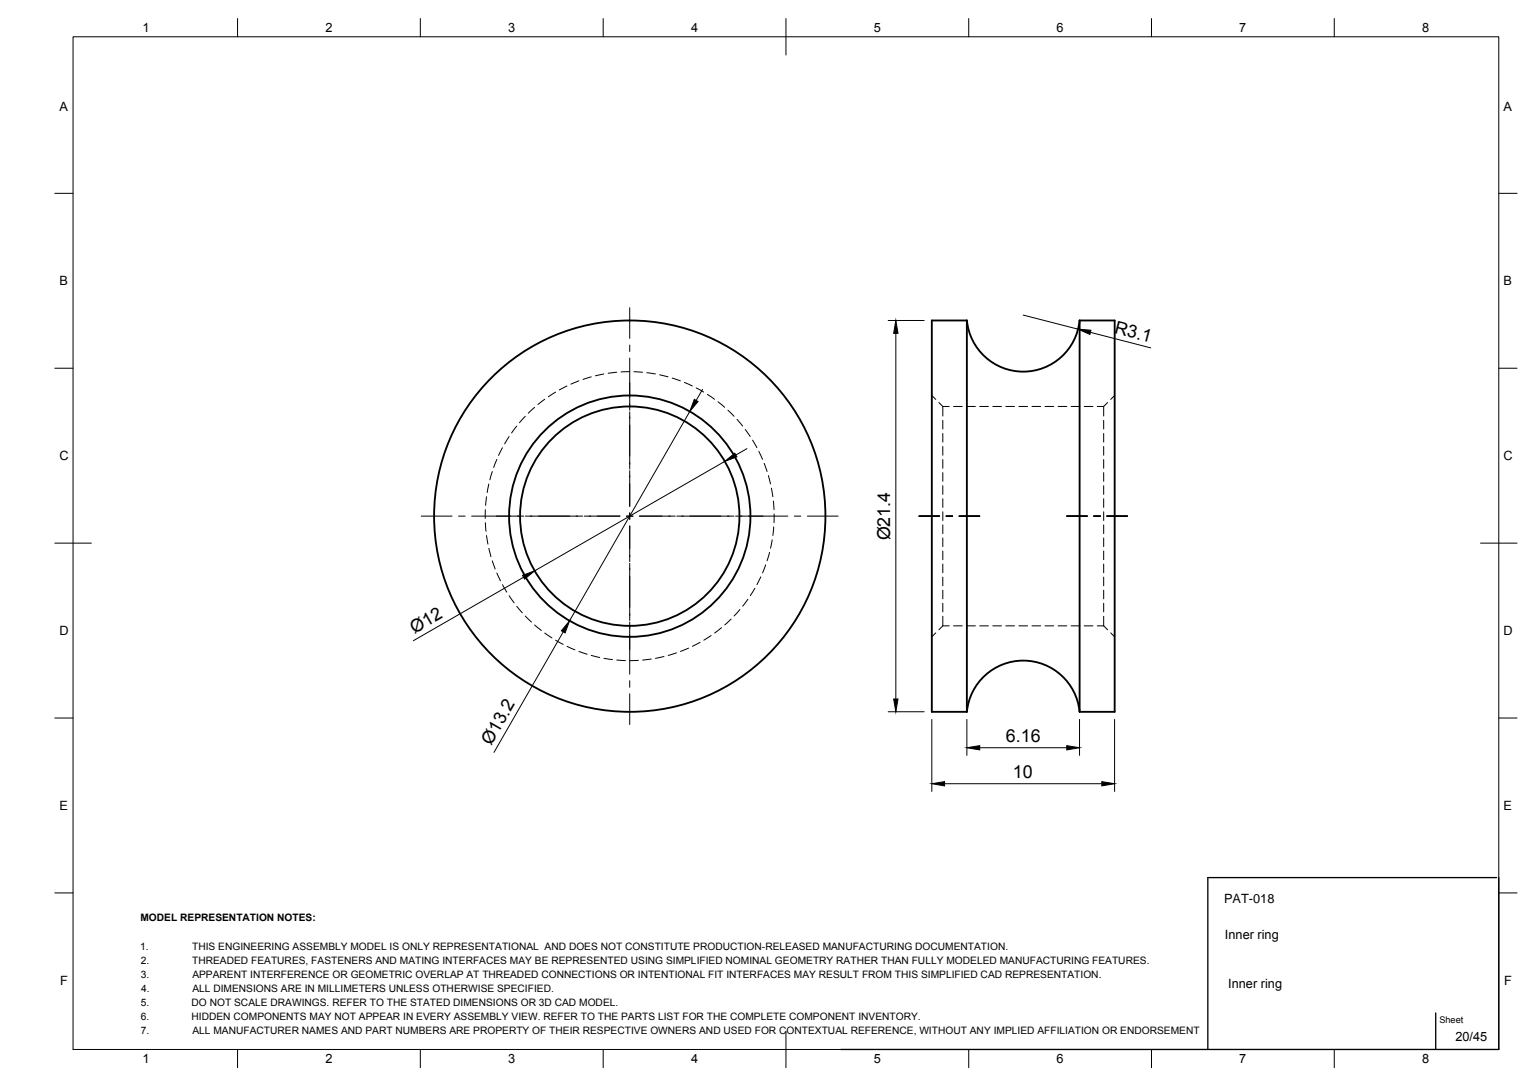
ISO-10303-21;
HEADER;
/* Generated by software containing ST-Developer
 * from STEP Tools, Inc. (www.steptools.com) 
 */

FILE_DESCRIPTION(
/* description */ ('Cam-driven reciprocating slide'),
/* implementation_level */ '2;1');

FILE_NAME(
/* name */ 'Inner ring.step',
/* time_stamp */ '2026-10-28T03:25:20-07:00',
/* author */ (''),
/* organization */ (''),
/* preprocessor_version */ 'ST-DEVELOPER v20.2',
/* originating_system */ 'Autodesk Translation Framework v15.17.0.0',
/* authorisation */ '');

FILE_SCHEMA (('AUTOMOTIVE_DESIGN { 1 0 10303 214 3 1 1 }'));
ENDSEC;

DATA;
#10=MECHANICAL_DESIGN_GEOMETRIC_PRESENTATION_REPRESENTATION('',(#435),#13277);
#315=CONICAL_SURFACE('',#7167,0.63,0.785398163397448);
#316=CONICAL_SURFACE('',#7174,0.63,0.785398163397448);
#330=TOROIDAL_SURFACE('',#7156,1.1,0.309556);
#361=SHAPE_REPRESENTATION_RELATIONSHIP('SRR','None',#13455,#398);
#398=ADVANCED_BREP_SHAPE_REPRESENTATION('',(#479),#13250);
#435=STYLED_ITEM('',(#13720),#479);
#479=MANIFOLD_SOLID_BREP('Body1',#6411);
#618=FACE_BOUND('',#1547,.T.);
#619=FACE_BOUND('',#1550,.T.);
#764=PLANE('',#7169);
#765=PLANE('',#7172);
#1052=FACE_OUTER_BOUND('',#1542,.T.);
#1053=FACE_OUTER_BOUND('',#1543,.T.);
#1054=FACE_OUTER_BOUND('',#1544,.T.);
#1055=FACE_OUTER_BOUND('',#1545,.T.);
#1056=FACE_OUTER_BOUND('',#1546,.T.);
#1057=FACE_OUTER_BOUND('',#1548,.T.);
#1058=FACE_OUTER_BOUND('',#1549,.T.);
#1059=FACE_OUTER_BOUND('',#1551,.T.);
#1542=EDGE_LOOP('',(#5008,#5009,#5010,#5011,#5012,#5013));
#1543=EDGE_LOOP('',(#5014,#5015,#5016,#5017,#5018));
#1544=EDGE_LOOP('',(#5019,#5020,#5021,#5022));
#1545=EDGE_LOOP('',(#5023,#5024,#5025,#5026));
#1546=EDGE_LOOP('',(#5027));
#1547=EDGE_LOOP('',(#5028));
#1548=EDGE_LOOP('',(#5029,#5030,#5031,#5032,#5033));
#1549=EDGE_LOOP('',(#5034));
#1550=EDGE_LOOP('',(#5035));
#1551=EDGE_LOOP('',(#5036,#5037,#5038,#5039));
#2032=LINE('',#11842,#2471);
#2033=LINE('',#11848,#2472);
#2034=LINE('',#11852,#2473);
#2035=LINE('',#11858,#2474);
#2036=LINE('',#11863,#2475);
#2471=VECTOR('',#8488,1.070235);
#2472=VECTOR('',#8495,0.6);
#2473=VECTOR('',#8500,0.63);
#2474=VECTOR('',#8509,1.070235);
#2475=VECTOR('',#8516,0.63);
#2847=CIRCLE('',#7157,1.070235);
#2848=CIRCLE('',#7158,1.070235);
#2849=CIRCLE('',#7159,0.309556);
#2850=CIRCLE('',#7160,1.070235);
#2851=CIRCLE('',#7161,1.070235);
#2852=CIRCLE('',#7163,1.070235);
#2853=CIRCLE('',#7165,0.6);
#2854=CIRCLE('',#7166,0.6);
#2855=CIRCLE('',#7168,0.66);
#2856=CIRCLE('',#7171,1.070235);
#2857=CIRCLE('',#7173,0.66);
#3259=VERTEX_POINT('',#11831);
#3260=VERTEX_POINT('',#11832);
#3261=VERTEX_POINT('',#11835);
#3262=VERTEX_POINT('',#11837);
#3263=VERTEX_POINT('',#11841);
#3264=VERTEX_POINT('',#11845);
#3265=VERTEX_POINT('',#11847);
#3266=VERTEX_POINT('',#11851);
#3267=VERTEX_POINT('',#11856);
#3268=VERTEX_POINT('',#11860);
#3894=EDGE_CURVE('',#3259,#3260,#2847,.T.);
#3895=EDGE_CURVE('',#3260,#3259,#2848,.T.);
#3896=EDGE_CURVE('',#3260,#3261,#2849,.T.);
#3897=EDGE_CURVE('',#3262,#3261,#2850,.T.);
#3898=EDGE_CURVE('',#3261,#3262,#2851,.T.);
#3899=EDGE_CURVE('',#3262,#3263,#2032,.T.);
#3900=EDGE_CURVE('',#3263,#3263,#2852,.T.);
#3901=EDGE_CURVE('',#3264,#3264,#2853,.T.);
#3902=EDGE_CURVE('',#3264,#3265,#2033,.T.);
#3903=EDGE_CURVE('',#3265,#3265,#2854,.T.);
#3904=EDGE_CURVE('',#3265,#3266,#2034,.T.);
#3905=EDGE_CURVE('',#3266,#3266,#2855,.T.);
#3906=EDGE_CURVE('',#3267,#3267,#2856,.T.);
#3907=EDGE_CURVE('',#3267,#3259,#2035,.T.);
#3908=EDGE_CURVE('',#3268,#3268,#2857,.T.);
#3909=EDGE_CURVE('',#3268,#3264,#2036,.T.);
#5008=ORIENTED_EDGE('',*,*,#3894,.F.);
#5009=ORIENTED_EDGE('',*,*,#3895,.F.);
#5010=ORIENTED_EDGE('',*,*,#3896,.T.);
#5011=ORIENTED_EDGE('',*,*,#3897,.F.);
#5012=ORIENTED_EDGE('',*,*,#3898,.F.);
#5013=ORIENTED_EDGE('',*,*,#3896,.F.);
#5014=ORIENTED_EDGE('',*,*,#3897,.T.);
#5015=ORIENTED_EDGE('',*,*,#3898,.T.);
#5016=ORIENTED_EDGE('',*,*,#3899,.T.);
#5017=ORIENTED_EDGE('',*,*,#3900,.T.);
#5018=ORIENTED_EDGE('',*,*,#3899,.F.);
#5019=ORIENTED_EDGE('',*,*,#3901,.T.);
#5020=ORIENTED_EDGE('',*,*,#3902,.T.);
#5021=ORIENTED_EDGE('',*,*,#3903,.F.);
#5022=ORIENTED_EDGE('',*,*,#3902,.F.);
#5023=ORIENTED_EDGE('',*,*,#3903,.T.);
#5024=ORIENTED_EDGE('',*,*,#3904,.T.);
#5025=ORIENTED_EDGE('',*,*,#3905,.F.);
#5026=ORIENTED_EDGE('',*,*,#3904,.F.);
#5027=ORIENTED_EDGE('',*,*,#3900,.F.);
#5028=ORIENTED_EDGE('',*,*,#3905,.T.);
#5029=ORIENTED_EDGE('',*,*,#3906,.F.);
#5030=ORIENTED_EDGE('',*,*,#3907,.T.);
#5031=ORIENTED_EDGE('',*,*,#3894,.T.);
#5032=ORIENTED_EDGE('',*,*,#3895,.T.);
#5033=ORIENTED_EDGE('',*,*,#3907,.F.);
#5034=ORIENTED_EDGE('',*,*,#3906,.T.);
#5035=ORIENTED_EDGE('',*,*,#3908,.F.);
#5036=ORIENTED_EDGE('',*,*,#3908,.T.);
#5037=ORIENTED_EDGE('',*,*,#3909,.T.);
#5038=ORIENTED_EDGE('',*,*,#3901,.F.);
#5039=ORIENTED_EDGE('',*,*,#3909,.F.);
#5959=CYLINDRICAL_SURFACE('',#7162,1.070235);
#5960=CYLINDRICAL_SURFACE('',#7164,0.6);
#5961=CYLINDRICAL_SURFACE('',#7170,1.070235);
#6170=ADVANCED_FACE('',(#1052),#330,.F.);
#6171=ADVANCED_FACE('',(#1053),#5959,.T.);
#6172=ADVANCED_FACE('',(#1054),#5960,.F.);
#6173=ADVANCED_FACE('',(#1055),#315,.F.);
#6174=ADVANCED_FACE('',(#1056,#618),#764,.T.);
#6175=ADVANCED_FACE('',(#1057),#5961,.T.);
#6176=ADVANCED_FACE('',(#1058,#619),#765,.T.);
#6177=ADVANCED_FACE('',(#1059),#316,.F.);
#6411=CLOSED_SHELL('',(#6170,#6171,#6172,#6173,#6174,#6175,#6176,#6177));
#7155=AXIS2_PLACEMENT_3D('',#11829,#8472,#8473);
#7156=AXIS2_PLACEMENT_3D('',#11830,#8474,#8475);
#7157=AXIS2_PLACEMENT_3D('',#11833,#8476,#8477);
#7158=AXIS2_PLACEMENT_3D('',#11834,#8478,#8479);
#7159=AXIS2_PLACEMENT_3D('',#11836,#8480,#8481);
#7160=AXIS2_PLACEMENT_3D('',#11838,#8482,#8483);
#7161=AXIS2_PLACEMENT_3D('',#11839,#8484,#8485);
#7162=AXIS2_PLACEMENT_3D('',#11840,#8486,#8487);
#7163=AXIS2_PLACEMENT_3D('',#11843,#8489,#8490);
#7164=AXIS2_PLACEMENT_3D('',#11844,#8491,#8492);
#7165=AXIS2_PLACEMENT_3D('',#11846,#8493,#8494);
#7166=AXIS2_PLACEMENT_3D('',#11849,#8496,#8497);
#7167=AXIS2_PLACEMENT_3D('',#11850,#8498,#8499);
#7168=AXIS2_PLACEMENT_3D('',#11853,#8501,#8502);
#7169=AXIS2_PLACEMENT_3D('',#11854,#8503,#8504);
#7170=AXIS2_PLACEMENT_3D('',#11855,#8505,#8506);
#7171=AXIS2_PLACEMENT_3D('',#11857,#8507,#8508);
#7172=AXIS2_PLACEMENT_3D('',#11859,#8510,#8511);
#7173=AXIS2_PLACEMENT_3D('',#11861,#8512,#8513);
#7174=AXIS2_PLACEMENT_3D('',#11862,#8514,#8515);
#8472=DIRECTION('axis',(0.,0.,1.));
#8473=DIRECTION('refdir',(1.,0.,0.));
#8474=DIRECTION('center_axis',(0.,-1.,0.));
#8475=DIRECTION('ref_axis',(0.,0.,-1.));
#8476=DIRECTION('center_axis',(0.,-1.,0.));
#8477=DIRECTION('ref_axis',(1.,0.,0.));
#8478=DIRECTION('center_axis',(0.,-1.,0.));
#8479=DIRECTION('ref_axis',(1.,0.,0.));
#8480=DIRECTION('center_axis',(1.,0.,1.22464679914735E-16));
#8481=DIRECTION('ref_axis',(-1.22464679914735E-16,0.,1.));
#8482=DIRECTION('center_axis',(0.,1.,0.));
#8483=DIRECTION('ref_axis',(1.,0.,0.));
#8484=DIRECTION('center_axis',(0.,1.,0.));
#8485=DIRECTION('ref_axis',(1.,0.,0.));
#8486=DIRECTION('center_axis',(0.,-1.,0.));
#8487=DIRECTION('ref_axis',(1.,0.,0.));
#8488=DIRECTION('',(0.,1.,0.));
#8489=DIRECTION('center_axis',(0.,-1.,0.));
#8490=DIRECTION('ref_axis',(1.,0.,0.));
#8491=DIRECTION('center_axis',(0.,-1.,0.));
#8492=DIRECTION('ref_axis',(1.,0.,0.));
#8493=DIRECTION('center_axis',(0.,-1.,0.));
#8494=DIRECTION('ref_axis',(1.,0.,0.));
#8495=DIRECTION('',(0.,1.,0.));
#8496=DIRECTION('center_axis',(0.,-1.,0.));
#8497=DIRECTION('ref_axis',(1.,0.,0.));
#8498=DIRECTION('center_axis',(0.,1.,0.));
#8499=DIRECTION('ref_axis',(1.,0.,0.));
#8500=DIRECTION('',(-0.707106781186548,0.707106781186547,-8.65956056235493E-17));
#8501=DIRECTION('center_axis',(0.,-1.,0.));
#8502=DIRECTION('ref_axis',(1.,0.,0.));
#8503=DIRECTION('center_axis',(0.,1.,0.));
#8504=DIRECTION('ref_axis',(0.,0.,1.));
#8505=DIRECTION('center_axis',(0.,-1.,0.));
#8506=DIRECTION('ref_axis',(1.,0.,0.));
#8507=DIRECTION('center_axis',(0.,-1.,0.));
#8508=DIRECTION('ref_axis',(1.,0.,0.));
#8509=DIRECTION('',(0.,1.,0.));
#8510=DIRECTION('center_axis',(0.,-1.,0.));
#8511=DIRECTION('ref_axis',(0.,0.,-1.));
#8512=DIRECTION('center_axis',(0.,-1.,0.));
#8513=DIRECTION('ref_axis',(1.,0.,0.));
#8514=DIRECTION('center_axis',(0.,-1.,0.));
#8515=DIRECTION('ref_axis',(1.,0.,0.));
#8516=DIRECTION('',(0.707106781186548,0.707106781186547,8.65956056235493E-17));
#11829=CARTESIAN_POINT('',(0.,0.,0.));
#11830=CARTESIAN_POINT('Origin',(0.,0.,0.));
#11831=CARTESIAN_POINT('',(-1.070235,-0.308121667383195,-1.31065986708547E-16));
#11832=CARTESIAN_POINT('',(-1.31065986708547E-16,-0.308121667383195,1.070235));
#11833=CARTESIAN_POINT('Origin',(0.,-0.308121667383195,0.));
#11834=CARTESIAN_POINT('Origin',(0.,-0.308121667383195,0.));
#11835=CARTESIAN_POINT('',(-1.31065986708547E-16,0.308121667383195,1.070235));
#11836=CARTESIAN_POINT('Origin',(-1.34711147906209E-16,0.,1.1));
#11837=CARTESIAN_POINT('',(-1.070235,0.308121667383195,1.31065986708547E-16));
#11838=CARTESIAN_POINT('Origin',(0.,0.308121667383195,0.));
#11839=CARTESIAN_POINT('Origin',(0.,0.308121667383195,0.));
#11840=CARTESIAN_POINT('Origin',(0.,0.,0.));
#11841=CARTESIAN_POINT('',(-1.070235,0.5,-1.31065986708547E-16));
#11842=CARTESIAN_POINT('',(-1.070235,0.,-1.31065986708547E-16));
#11843=CARTESIAN_POINT('Origin',(0.,0.5,0.));
#11844=CARTESIAN_POINT('Origin',(0.,0.,0.));
#11845=CARTESIAN_POINT('',(-0.6,-0.44,-7.34788079488412E-17));
#11846=CARTESIAN_POINT('Origin',(0.,-0.44,0.));
#11847=CARTESIAN_POINT('',(-0.6,0.44,-7.34788079488412E-17));
#11848=CARTESIAN_POINT('',(-0.6,0.,-7.34788079488412E-17));
#11849=CARTESIAN_POINT('Origin',(0.,0.44,0.));
#11850=CARTESIAN_POINT('Origin',(0.,0.47,0.));
#11851=CARTESIAN_POINT('',(-0.66,0.5,-8.08266887437253E-17));
#11852=CARTESIAN_POINT('',(-0.63,0.47,-7.71527483462832E-17));
#11853=CARTESIAN_POINT('Origin',(0.,0.5,0.));
#11854=CARTESIAN_POINT('Origin',(1.070235,0.5,0.));
#11855=CARTESIAN_POINT('Origin',(0.,0.,0.));
#11856=CARTESIAN_POINT('',(-1.070235,-0.5,-1.31065986708547E-16));
#11857=CARTESIAN_POINT('Origin',(0.,-0.5,0.));
#11858=CARTESIAN_POINT('',(-1.070235,0.,-1.31065986708547E-16));
#11859=CARTESIAN_POINT('Origin',(0.66,-0.5,0.));
#11860=CARTESIAN_POINT('',(-0.66,-0.5,-8.08266887437253E-17));
#11861=CARTESIAN_POINT('Origin',(0.,-0.5,0.));
#11862=CARTESIAN_POINT('Origin',(0.,-0.47,0.));
#11863=CARTESIAN_POINT('',(-0.63,-0.47,-7.71527483462832E-17));
#13206=UNCERTAINTY_MEASURE_WITH_UNIT(LENGTH_MEASURE(0.001),#13278,
'DISTANCE_ACCURACY_VALUE',
'Maximum model space distance between geometric entities at asserted c
onnectivities');
#13233=UNCERTAINTY_MEASURE_WITH_UNIT(LENGTH_MEASURE(0.001),#13278,
'DISTANCE_ACCURACY_VALUE',
'Maximum model space distance between geometric entities at asserted c
onnectivities');
#13250=(
GEOMETRIC_REPRESENTATION_CONTEXT(3)
GLOBAL_UNCERTAINTY_ASSIGNED_CONTEXT((#13206))
GLOBAL_UNIT_ASSIGNED_CONTEXT((#13278,#13280,#13281))
REPRESENTATION_CONTEXT('','3D')
);
#13277=(
GEOMETRIC_REPRESENTATION_CONTEXT(3)
GLOBAL_UNCERTAINTY_ASSIGNED_CONTEXT((#13233))
GLOBAL_UNIT_ASSIGNED_CONTEXT((#13278,#13280,#13281))
REPRESENTATION_CONTEXT('','3D')
);
#13278=(
LENGTH_UNIT()
NAMED_UNIT(*)
SI_UNIT(.CENTI.,.METRE.)
);
#13280=(
NAMED_UNIT(*)
PLANE_ANGLE_UNIT()
SI_UNIT($,.RADIAN.)
);
#13281=(
NAMED_UNIT(*)
SI_UNIT($,.STERADIAN.)
SOLID_ANGLE_UNIT()
);
#13298=SHAPE_DEFINITION_REPRESENTATION(#13341,#13455);
#13341=PRODUCT_DEFINITION_SHAPE('',$,#13499);
#13455=SHAPE_REPRESENTATION('',(#7155),#13250);
#13482=PRODUCT_DEFINITION_CONTEXT('part definition',#13613,'design');
#13499=PRODUCT_DEFINITION('Inner ring','Inner ring',#13542,#13482);
#13542=PRODUCT_DEFINITION_FORMATION('',$,#13631);
#13613=APPLICATION_CONTEXT(
'Core Data for Automotive Mechanical Design Process');
#13614=PRODUCT_CONTEXT('part definition',#13613,'mechanical');
#13631=PRODUCT('Inner ring','Inner ring','Inner ring',(#13614));
#13714=COLOUR_RGB('Grey',0.48,0.52,0.57);
#13715=FILL_AREA_STYLE_COLOUR('',#13714);
#13716=FILL_AREA_STYLE('',(#13715));
#13717=SURFACE_STYLE_FILL_AREA(#13716);
#13718=SURFACE_SIDE_STYLE('',(#13717));
#13719=SURFACE_STYLE_USAGE(.BOTH.,#13718);
#13720=PRESENTATION_STYLE_ASSIGNMENT((#13719));
ENDSEC;
END-ISO-10303-21;
